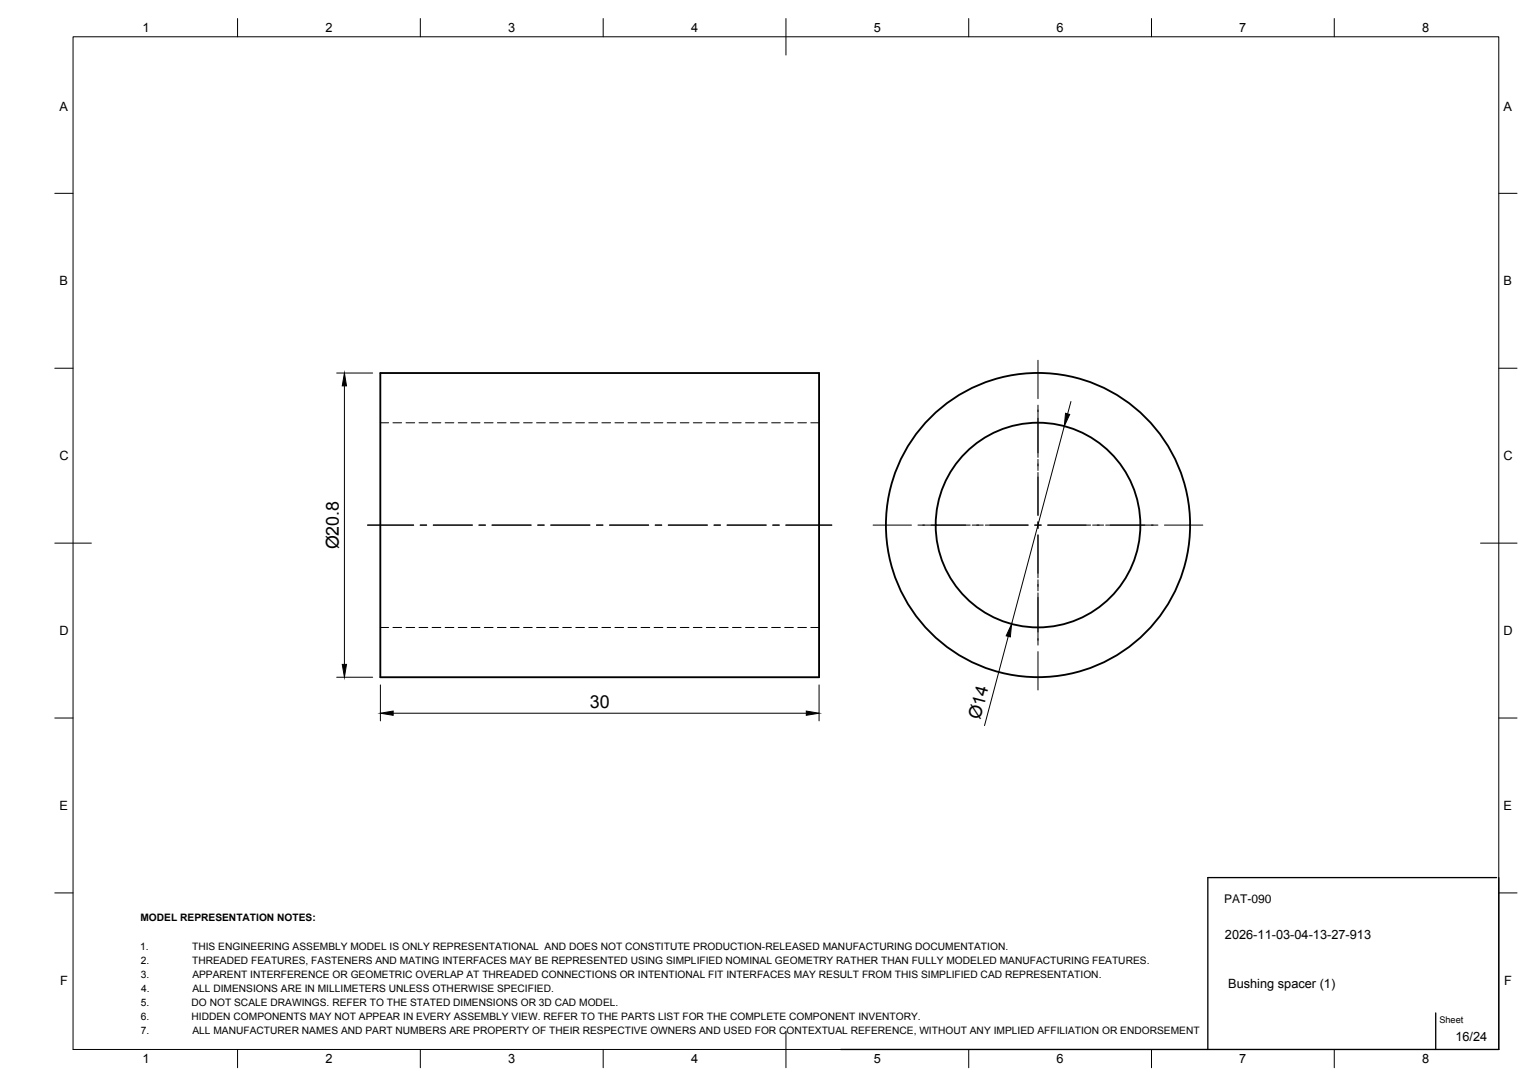
ISO-10303-21;
HEADER;
/* Generated by software containing ST-Developer
 * from STEP Tools, Inc. (www.steptools.com) 
 */

FILE_DESCRIPTION(
/* description */ ('Round-Shaft Linear Stage with Ball Bushings'),
/* implementation_level */ '2;1');

FILE_NAME(
/* name */ 'Bushing spacer (1).step',
/* time_stamp */ '2026-10-27T10:47:55-07:00',
/* author */ (''),
/* organization */ (''),
/* preprocessor_version */ 'ST-DEVELOPER v20.2',
/* originating_system */ 'Autodesk Translation Framework v15.17.0.0',
/* authorisation */ '');

FILE_SCHEMA (('AUTOMOTIVE_DESIGN { 1 0 10303 214 3 1 1 }'));
ENDSEC;

DATA;
#10=MECHANICAL_DESIGN_GEOMETRIC_PRESENTATION_REPRESENTATION('',(#312),#7835);
#270=SHAPE_REPRESENTATION_RELATIONSHIP('SRR','None',#7959,#291);
#291=ADVANCED_BREP_SHAPE_REPRESENTATION('',(#332),#7823);
#312=STYLED_ITEM('',(#8158),#332);
#332=MANIFOLD_SOLID_BREP('Body1',#4403);
#405=FACE_BOUND('',#1075,.T.);
#406=FACE_BOUND('',#1077,.T.);
#542=PLANE('',#4900);
#543=PLANE('',#4901);
#750=FACE_OUTER_BOUND('',#1072,.T.);
#751=FACE_OUTER_BOUND('',#1073,.T.);
#752=FACE_OUTER_BOUND('',#1074,.T.);
#753=FACE_OUTER_BOUND('',#1076,.T.);
#1072=EDGE_LOOP('',(#3554,#3555,#3556,#3557));
#1073=EDGE_LOOP('',(#3558,#3559,#3560,#3561));
#1074=EDGE_LOOP('',(#3562));
#1075=EDGE_LOOP('',(#3563));
#1076=EDGE_LOOP('',(#3564));
#1077=EDGE_LOOP('',(#3565));
#1432=LINE('',#7187,#1772);
#1433=LINE('',#7193,#1773);
#1772=VECTOR('',#5853,0.7);
#1773=VECTOR('',#5860,1.04);
#2026=CIRCLE('',#4895,0.7);
#2027=CIRCLE('',#4896,0.7);
#2028=CIRCLE('',#4898,1.04);
#2029=CIRCLE('',#4899,1.04);
#2303=VERTEX_POINT('',#7184);
#2304=VERTEX_POINT('',#7186);
#2305=VERTEX_POINT('',#7190);
#2306=VERTEX_POINT('',#7192);
#2745=EDGE_CURVE('',#2303,#2303,#2026,.T.);
#2746=EDGE_CURVE('',#2303,#2304,#1432,.T.);
#2747=EDGE_CURVE('',#2304,#2304,#2027,.T.);
#2748=EDGE_CURVE('',#2305,#2305,#2028,.T.);
#2749=EDGE_CURVE('',#2305,#2306,#1433,.T.);
#2750=EDGE_CURVE('',#2306,#2306,#2029,.T.);
#3554=ORIENTED_EDGE('',*,*,#2745,.F.);
#3555=ORIENTED_EDGE('',*,*,#2746,.T.);
#3556=ORIENTED_EDGE('',*,*,#2747,.T.);
#3557=ORIENTED_EDGE('',*,*,#2746,.F.);
#3558=ORIENTED_EDGE('',*,*,#2748,.F.);
#3559=ORIENTED_EDGE('',*,*,#2749,.T.);
#3560=ORIENTED_EDGE('',*,*,#2750,.T.);
#3561=ORIENTED_EDGE('',*,*,#2749,.F.);
#3562=ORIENTED_EDGE('',*,*,#2748,.T.);
#3563=ORIENTED_EDGE('',*,*,#2745,.T.);
#3564=ORIENTED_EDGE('',*,*,#2750,.F.);
#3565=ORIENTED_EDGE('',*,*,#2747,.F.);
#4098=CYLINDRICAL_SURFACE('',#4894,0.7);
#4099=CYLINDRICAL_SURFACE('',#4897,1.04);
#4269=ADVANCED_FACE('',(#750),#4098,.F.);
#4270=ADVANCED_FACE('',(#751),#4099,.T.);
#4271=ADVANCED_FACE('',(#752,#405),#542,.T.);
#4272=ADVANCED_FACE('',(#753,#406),#543,.F.);
#4403=CLOSED_SHELL('',(#4269,#4270,#4271,#4272));
#4893=AXIS2_PLACEMENT_3D('',#7182,#5847,#5848);
#4894=AXIS2_PLACEMENT_3D('',#7183,#5849,#5850);
#4895=AXIS2_PLACEMENT_3D('',#7185,#5851,#5852);
#4896=AXIS2_PLACEMENT_3D('',#7188,#5854,#5855);
#4897=AXIS2_PLACEMENT_3D('',#7189,#5856,#5857);
#4898=AXIS2_PLACEMENT_3D('',#7191,#5858,#5859);
#4899=AXIS2_PLACEMENT_3D('',#7194,#5861,#5862);
#4900=AXIS2_PLACEMENT_3D('',#7195,#5863,#5864);
#4901=AXIS2_PLACEMENT_3D('',#7196,#5865,#5866);
#5847=DIRECTION('axis',(0.,0.,1.));
#5848=DIRECTION('refdir',(1.,0.,0.));
#5849=DIRECTION('center_axis',(1.,0.,0.));
#5850=DIRECTION('ref_axis',(0.,0.,-1.));
#5851=DIRECTION('center_axis',(-1.,0.,0.));
#5852=DIRECTION('ref_axis',(0.,0.,-1.));
#5853=DIRECTION('',(-1.,0.,0.));
#5854=DIRECTION('center_axis',(-1.,0.,0.));
#5855=DIRECTION('ref_axis',(0.,0.,-1.));
#5856=DIRECTION('center_axis',(1.,0.,0.));
#5857=DIRECTION('ref_axis',(0.,0.,-1.));
#5858=DIRECTION('center_axis',(1.,0.,0.));
#5859=DIRECTION('ref_axis',(0.,0.,-1.));
#5860=DIRECTION('',(-1.,0.,0.));
#5861=DIRECTION('center_axis',(1.,0.,0.));
#5862=DIRECTION('ref_axis',(0.,0.,-1.));
#5863=DIRECTION('center_axis',(1.,0.,0.));
#5864=DIRECTION('ref_axis',(0.,0.,-1.));
#5865=DIRECTION('center_axis',(1.,0.,0.));
#5866=DIRECTION('ref_axis',(0.,0.,-1.));
#7182=CARTESIAN_POINT('',(0.,0.,0.));
#7183=CARTESIAN_POINT('Origin',(13.5,4.,3.3));
#7184=CARTESIAN_POINT('',(16.5,4.,4.));
#7185=CARTESIAN_POINT('Origin',(16.5,4.,3.3));
#7186=CARTESIAN_POINT('',(13.5,4.,4.));
#7187=CARTESIAN_POINT('',(13.5,4.,4.));
#7188=CARTESIAN_POINT('Origin',(13.5,4.,3.3));
#7189=CARTESIAN_POINT('Origin',(13.5,4.,3.3));
#7190=CARTESIAN_POINT('',(16.5,4.,4.34));
#7191=CARTESIAN_POINT('Origin',(16.5,4.,3.3));
#7192=CARTESIAN_POINT('',(13.5,4.,4.34));
#7193=CARTESIAN_POINT('',(13.5,4.,4.34));
#7194=CARTESIAN_POINT('Origin',(13.5,4.,3.3));
#7195=CARTESIAN_POINT('Origin',(16.5,4.,3.3));
#7196=CARTESIAN_POINT('Origin',(13.5,4.,3.3));
#7797=UNCERTAINTY_MEASURE_WITH_UNIT(LENGTH_MEASURE(0.001),#7836,
'DISTANCE_ACCURACY_VALUE',
'Maximum model space distance between geometric entities at asserted c
onnectivities');
#7809=UNCERTAINTY_MEASURE_WITH_UNIT(LENGTH_MEASURE(0.001),#7836,
'DISTANCE_ACCURACY_VALUE',
'Maximum model space distance between geometric entities at asserted c
onnectivities');
#7823=(
GEOMETRIC_REPRESENTATION_CONTEXT(3)
GLOBAL_UNCERTAINTY_ASSIGNED_CONTEXT((#7797))
GLOBAL_UNIT_ASSIGNED_CONTEXT((#7836,#7838,#7839))
REPRESENTATION_CONTEXT('','3D')
);
#7835=(
GEOMETRIC_REPRESENTATION_CONTEXT(3)
GLOBAL_UNCERTAINTY_ASSIGNED_CONTEXT((#7809))
GLOBAL_UNIT_ASSIGNED_CONTEXT((#7836,#7838,#7839))
REPRESENTATION_CONTEXT('','3D')
);
#7836=(
LENGTH_UNIT()
NAMED_UNIT(*)
SI_UNIT(.CENTI.,.METRE.)
);
#7838=(
NAMED_UNIT(*)
PLANE_ANGLE_UNIT()
SI_UNIT($,.RADIAN.)
);
#7839=(
NAMED_UNIT(*)
SI_UNIT($,.STERADIAN.)
SOLID_ANGLE_UNIT()
);
#7853=SHAPE_DEFINITION_REPRESENTATION(#7878,#7959);
#7878=PRODUCT_DEFINITION_SHAPE('',$,#7985);
#7959=SHAPE_REPRESENTATION('',(#4893),#7823);
#7971=PRODUCT_DEFINITION_CONTEXT('part definition',#8048,'design');
#7985=PRODUCT_DEFINITION('Bushing spacer (1)','Bushing spacer (1)',#8010,
#7971);
#8010=PRODUCT_DEFINITION_FORMATION('',$,#8063);
#8048=APPLICATION_CONTEXT(
'Core Data for Automotive Mechanical Design Process');
#8049=PRODUCT_CONTEXT('part definition',#8048,'mechanical');
#8063=PRODUCT('Bushing spacer (1)','Bushing spacer (1)','Bushing spacer (1)',
(#8049));
#8152=COLOUR_RGB('Off White',0.89,0.88,0.83);
#8153=FILL_AREA_STYLE_COLOUR('',#8152);
#8154=FILL_AREA_STYLE('',(#8153));
#8155=SURFACE_STYLE_FILL_AREA(#8154);
#8156=SURFACE_SIDE_STYLE('',(#8155));
#8157=SURFACE_STYLE_USAGE(.BOTH.,#8156);
#8158=PRESENTATION_STYLE_ASSIGNMENT((#8157));
ENDSEC;
END-ISO-10303-21;
